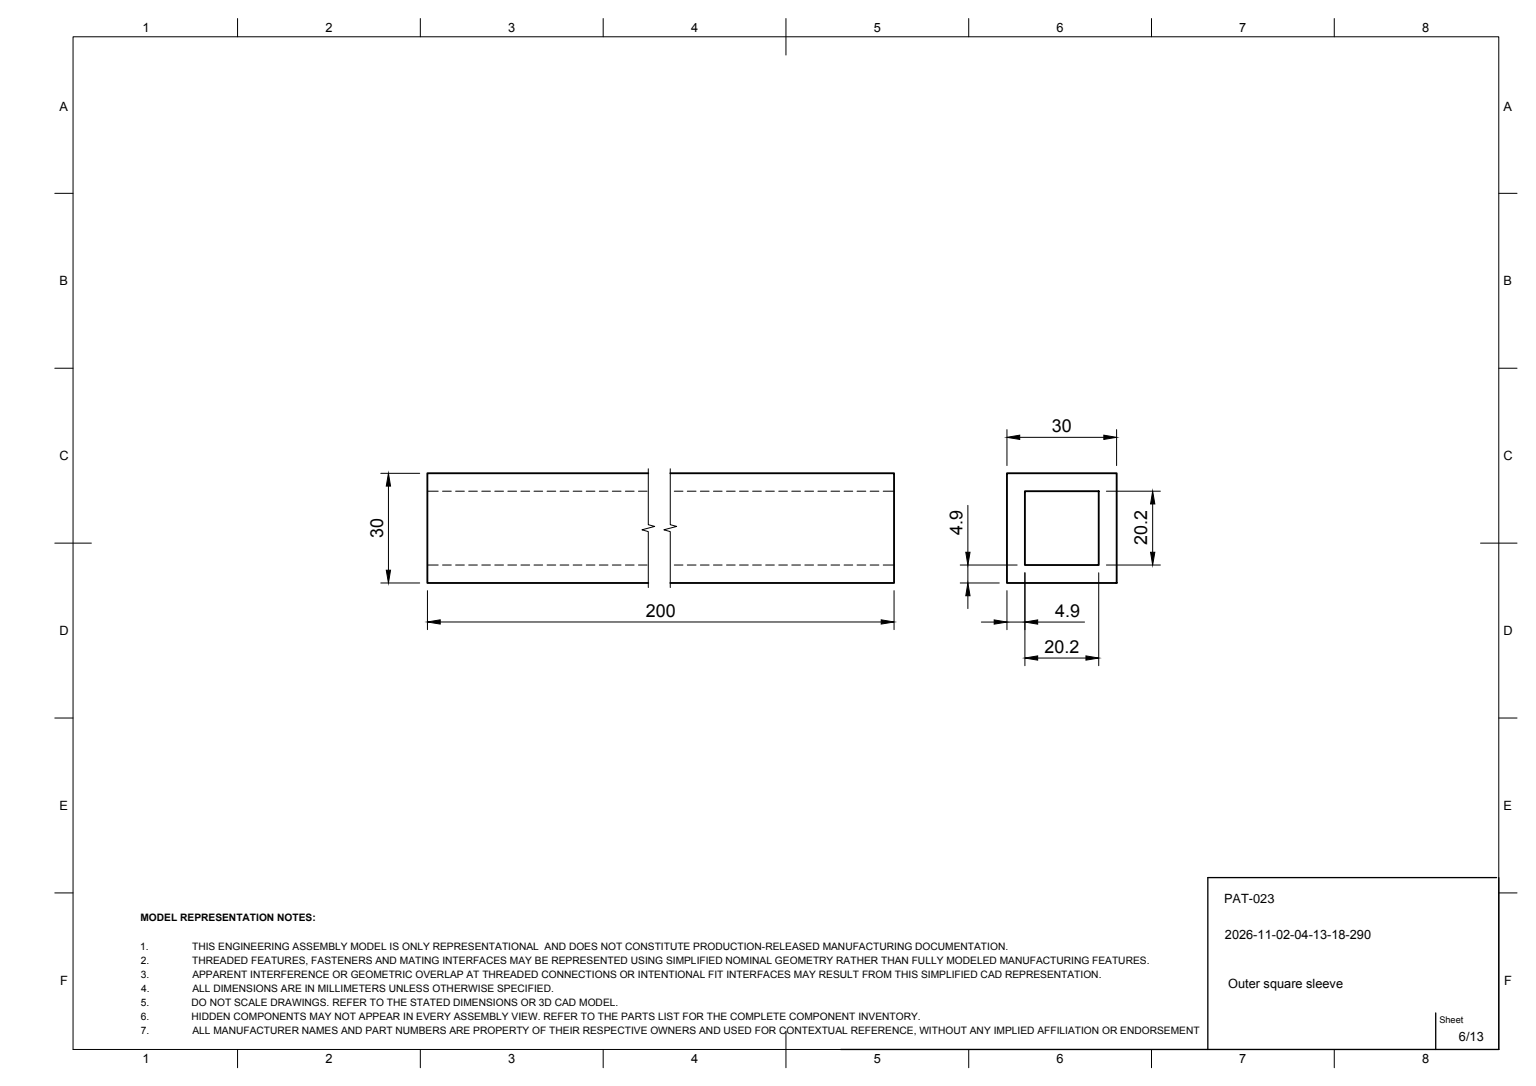
ISO-10303-21;
HEADER;
/* Generated by software containing ST-Developer
 * from STEP Tools, Inc. (www.steptools.com) 
 */

FILE_DESCRIPTION(
/* description */ ('PAT-023'),
/* implementation_level */ '2;1');

FILE_NAME(
/* name */ 'Outer square sleeve.step',
/* time_stamp */ '2026-10-29T15:47:46-07:00',
/* author */ (''),
/* organization */ (''),
/* preprocessor_version */ 'ST-DEVELOPER v20.2',
/* originating_system */ 'Autodesk Translation Framework v15.17.0.0',
/* authorisation */ '');

FILE_SCHEMA (('AUTOMOTIVE_DESIGN { 1 0 10303 214 3 1 1 }'));
ENDSEC;

DATA;
#10=MECHANICAL_DESIGN_GEOMETRIC_PRESENTATION_REPRESENTATION('',(#85),#3773);
#69=SHAPE_REPRESENTATION_RELATIONSHIP('SRR','None',#3816,#77);
#77=ADVANCED_BREP_SHAPE_REPRESENTATION('',(#93),#3764);
#85=STYLED_ITEM('',(#3939),#93);
#93=MANIFOLD_SOLID_BREP('Body1',#2238);
#102=FACE_BOUND('',#355,.T.);
#103=FACE_BOUND('',#357,.T.);
#121=PLANE('',#2347);
#122=PLANE('',#2348);
#123=PLANE('',#2349);
#124=PLANE('',#2350);
#125=PLANE('',#2351);
#126=PLANE('',#2352);
#127=PLANE('',#2353);
#128=PLANE('',#2354);
#129=PLANE('',#2355);
#130=PLANE('',#2356);
#225=FACE_OUTER_BOUND('',#346,.T.);
#226=FACE_OUTER_BOUND('',#347,.T.);
#227=FACE_OUTER_BOUND('',#348,.T.);
#228=FACE_OUTER_BOUND('',#349,.T.);
#229=FACE_OUTER_BOUND('',#350,.T.);
#230=FACE_OUTER_BOUND('',#351,.T.);
#231=FACE_OUTER_BOUND('',#352,.T.);
#232=FACE_OUTER_BOUND('',#353,.T.);
#233=FACE_OUTER_BOUND('',#354,.T.);
#234=FACE_OUTER_BOUND('',#356,.T.);
#346=EDGE_LOOP('',(#1547,#1548,#1549,#1550));
#347=EDGE_LOOP('',(#1551,#1552,#1553,#1554));
#348=EDGE_LOOP('',(#1555,#1556,#1557,#1558));
#349=EDGE_LOOP('',(#1559,#1560,#1561,#1562));
#350=EDGE_LOOP('',(#1563,#1564,#1565,#1566));
#351=EDGE_LOOP('',(#1567,#1568,#1569,#1570));
#352=EDGE_LOOP('',(#1571,#1572,#1573,#1574));
#353=EDGE_LOOP('',(#1575,#1576,#1577,#1578));
#354=EDGE_LOOP('',(#1579,#1580,#1581,#1582));
#355=EDGE_LOOP('',(#1583,#1584,#1585,#1586));
#356=EDGE_LOOP('',(#1587,#1588,#1589,#1590));
#357=EDGE_LOOP('',(#1591,#1592,#1593,#1594));
#484=LINE('',#3141,#748);
#485=LINE('',#3143,#749);
#486=LINE('',#3145,#750);
#487=LINE('',#3146,#751);
#488=LINE('',#3149,#752);
#489=LINE('',#3151,#753);
#490=LINE('',#3152,#754);
#491=LINE('',#3155,#755);
#492=LINE('',#3157,#756);
#493=LINE('',#3158,#757);
#494=LINE('',#3160,#758);
#495=LINE('',#3161,#759);
#496=LINE('',#3165,#760);
#497=LINE('',#3167,#761);
#498=LINE('',#3169,#762);
#499=LINE('',#3170,#763);
#500=LINE('',#3173,#764);
#501=LINE('',#3175,#765);
#502=LINE('',#3176,#766);
#503=LINE('',#3179,#767);
#504=LINE('',#3181,#768);
#505=LINE('',#3182,#769);
#506=LINE('',#3184,#770);
#507=LINE('',#3185,#771);
#748=VECTOR('',#2543,1.);
#749=VECTOR('',#2544,1.);
#750=VECTOR('',#2545,1.);
#751=VECTOR('',#2546,1.);
#752=VECTOR('',#2549,1.);
#753=VECTOR('',#2550,1.);
#754=VECTOR('',#2551,1.);
#755=VECTOR('',#2554,1.);
#756=VECTOR('',#2555,1.);
#757=VECTOR('',#2556,1.);
#758=VECTOR('',#2559,1.);
#759=VECTOR('',#2560,1.);
#760=VECTOR('',#2563,1.);
#761=VECTOR('',#2564,1.);
#762=VECTOR('',#2565,1.);
#763=VECTOR('',#2566,1.);
#764=VECTOR('',#2569,1.);
#765=VECTOR('',#2570,1.);
#766=VECTOR('',#2571,1.);
#767=VECTOR('',#2574,1.);
#768=VECTOR('',#2575,1.);
#769=VECTOR('',#2576,1.);
#770=VECTOR('',#2579,1.);
#771=VECTOR('',#2580,1.);
#1035=VERTEX_POINT('',#3139);
#1036=VERTEX_POINT('',#3140);
#1037=VERTEX_POINT('',#3142);
#1038=VERTEX_POINT('',#3144);
#1039=VERTEX_POINT('',#3148);
#1040=VERTEX_POINT('',#3150);
#1041=VERTEX_POINT('',#3154);
#1042=VERTEX_POINT('',#3156);
#1043=VERTEX_POINT('',#3163);
#1044=VERTEX_POINT('',#3164);
#1045=VERTEX_POINT('',#3166);
#1046=VERTEX_POINT('',#3168);
#1047=VERTEX_POINT('',#3172);
#1048=VERTEX_POINT('',#3174);
#1049=VERTEX_POINT('',#3178);
#1050=VERTEX_POINT('',#3180);
#1236=EDGE_CURVE('',#1035,#1036,#484,.T.);
#1237=EDGE_CURVE('',#1037,#1035,#485,.T.);
#1238=EDGE_CURVE('',#1038,#1037,#486,.T.);
#1239=EDGE_CURVE('',#1038,#1036,#487,.T.);
#1240=EDGE_CURVE('',#1036,#1039,#488,.T.);
#1241=EDGE_CURVE('',#1040,#1038,#489,.T.);
#1242=EDGE_CURVE('',#1040,#1039,#490,.T.);
#1243=EDGE_CURVE('',#1039,#1041,#491,.T.);
#1244=EDGE_CURVE('',#1042,#1040,#492,.T.);
#1245=EDGE_CURVE('',#1042,#1041,#493,.T.);
#1246=EDGE_CURVE('',#1041,#1035,#494,.T.);
#1247=EDGE_CURVE('',#1037,#1042,#495,.T.);
#1248=EDGE_CURVE('',#1043,#1044,#496,.T.);
#1249=EDGE_CURVE('',#1044,#1045,#497,.T.);
#1250=EDGE_CURVE('',#1046,#1045,#498,.T.);
#1251=EDGE_CURVE('',#1043,#1046,#499,.T.);
#1252=EDGE_CURVE('',#1047,#1043,#500,.T.);
#1253=EDGE_CURVE('',#1048,#1046,#501,.T.);
#1254=EDGE_CURVE('',#1047,#1048,#502,.T.);
#1255=EDGE_CURVE('',#1049,#1047,#503,.T.);
#1256=EDGE_CURVE('',#1050,#1048,#504,.T.);
#1257=EDGE_CURVE('',#1049,#1050,#505,.T.);
#1258=EDGE_CURVE('',#1044,#1049,#506,.T.);
#1259=EDGE_CURVE('',#1045,#1050,#507,.T.);
#1547=ORIENTED_EDGE('',*,*,#1236,.F.);
#1548=ORIENTED_EDGE('',*,*,#1237,.F.);
#1549=ORIENTED_EDGE('',*,*,#1238,.F.);
#1550=ORIENTED_EDGE('',*,*,#1239,.T.);
#1551=ORIENTED_EDGE('',*,*,#1240,.F.);
#1552=ORIENTED_EDGE('',*,*,#1239,.F.);
#1553=ORIENTED_EDGE('',*,*,#1241,.F.);
#1554=ORIENTED_EDGE('',*,*,#1242,.T.);
#1555=ORIENTED_EDGE('',*,*,#1243,.F.);
#1556=ORIENTED_EDGE('',*,*,#1242,.F.);
#1557=ORIENTED_EDGE('',*,*,#1244,.F.);
#1558=ORIENTED_EDGE('',*,*,#1245,.T.);
#1559=ORIENTED_EDGE('',*,*,#1246,.F.);
#1560=ORIENTED_EDGE('',*,*,#1245,.F.);
#1561=ORIENTED_EDGE('',*,*,#1247,.F.);
#1562=ORIENTED_EDGE('',*,*,#1237,.T.);
#1563=ORIENTED_EDGE('',*,*,#1248,.T.);
#1564=ORIENTED_EDGE('',*,*,#1249,.T.);
#1565=ORIENTED_EDGE('',*,*,#1250,.F.);
#1566=ORIENTED_EDGE('',*,*,#1251,.F.);
#1567=ORIENTED_EDGE('',*,*,#1252,.T.);
#1568=ORIENTED_EDGE('',*,*,#1251,.T.);
#1569=ORIENTED_EDGE('',*,*,#1253,.F.);
#1570=ORIENTED_EDGE('',*,*,#1254,.F.);
#1571=ORIENTED_EDGE('',*,*,#1255,.T.);
#1572=ORIENTED_EDGE('',*,*,#1254,.T.);
#1573=ORIENTED_EDGE('',*,*,#1256,.F.);
#1574=ORIENTED_EDGE('',*,*,#1257,.F.);
#1575=ORIENTED_EDGE('',*,*,#1258,.T.);
#1576=ORIENTED_EDGE('',*,*,#1257,.T.);
#1577=ORIENTED_EDGE('',*,*,#1259,.F.);
#1578=ORIENTED_EDGE('',*,*,#1249,.F.);
#1579=ORIENTED_EDGE('',*,*,#1259,.T.);
#1580=ORIENTED_EDGE('',*,*,#1256,.T.);
#1581=ORIENTED_EDGE('',*,*,#1253,.T.);
#1582=ORIENTED_EDGE('',*,*,#1250,.T.);
#1583=ORIENTED_EDGE('',*,*,#1243,.T.);
#1584=ORIENTED_EDGE('',*,*,#1246,.T.);
#1585=ORIENTED_EDGE('',*,*,#1236,.T.);
#1586=ORIENTED_EDGE('',*,*,#1240,.T.);
#1587=ORIENTED_EDGE('',*,*,#1258,.F.);
#1588=ORIENTED_EDGE('',*,*,#1248,.F.);
#1589=ORIENTED_EDGE('',*,*,#1252,.F.);
#1590=ORIENTED_EDGE('',*,*,#1255,.F.);
#1591=ORIENTED_EDGE('',*,*,#1244,.T.);
#1592=ORIENTED_EDGE('',*,*,#1241,.T.);
#1593=ORIENTED_EDGE('',*,*,#1238,.T.);
#1594=ORIENTED_EDGE('',*,*,#1247,.T.);
#2125=ADVANCED_FACE('',(#225),#121,.F.);
#2126=ADVANCED_FACE('',(#226),#122,.F.);
#2127=ADVANCED_FACE('',(#227),#123,.F.);
#2128=ADVANCED_FACE('',(#228),#124,.F.);
#2129=ADVANCED_FACE('',(#229),#125,.T.);
#2130=ADVANCED_FACE('',(#230),#126,.T.);
#2131=ADVANCED_FACE('',(#231),#127,.T.);
#2132=ADVANCED_FACE('',(#232),#128,.T.);
#2133=ADVANCED_FACE('',(#233,#102),#129,.T.);
#2134=ADVANCED_FACE('',(#234,#103),#130,.F.);
#2238=CLOSED_SHELL('',(#2125,#2126,#2127,#2128,#2129,#2130,#2131,#2132,
#2133,#2134));
#2346=AXIS2_PLACEMENT_3D('',#3137,#2539,#2540);
#2347=AXIS2_PLACEMENT_3D('',#3138,#2541,#2542);
#2348=AXIS2_PLACEMENT_3D('',#3147,#2547,#2548);
#2349=AXIS2_PLACEMENT_3D('',#3153,#2552,#2553);
#2350=AXIS2_PLACEMENT_3D('',#3159,#2557,#2558);
#2351=AXIS2_PLACEMENT_3D('',#3162,#2561,#2562);
#2352=AXIS2_PLACEMENT_3D('',#3171,#2567,#2568);
#2353=AXIS2_PLACEMENT_3D('',#3177,#2572,#2573);
#2354=AXIS2_PLACEMENT_3D('',#3183,#2577,#2578);
#2355=AXIS2_PLACEMENT_3D('',#3186,#2581,#2582);
#2356=AXIS2_PLACEMENT_3D('',#3187,#2583,#2584);
#2539=DIRECTION('axis',(0.,0.,1.));
#2540=DIRECTION('refdir',(1.,0.,0.));
#2541=DIRECTION('center_axis',(0.,-1.,0.));
#2542=DIRECTION('ref_axis',(1.,0.,0.));
#2543=DIRECTION('',(-1.,0.,0.));
#2544=DIRECTION('',(0.,0.,1.));
#2545=DIRECTION('',(1.,0.,0.));
#2546=DIRECTION('',(0.,0.,1.));
#2547=DIRECTION('center_axis',(-1.,0.,0.));
#2548=DIRECTION('ref_axis',(0.,-1.,0.));
#2549=DIRECTION('',(0.,1.,0.));
#2550=DIRECTION('',(0.,-1.,0.));
#2551=DIRECTION('',(0.,0.,1.));
#2552=DIRECTION('center_axis',(0.,1.,0.));
#2553=DIRECTION('ref_axis',(-1.,0.,0.));
#2554=DIRECTION('',(1.,0.,0.));
#2555=DIRECTION('',(-1.,0.,0.));
#2556=DIRECTION('',(0.,0.,1.));
#2557=DIRECTION('center_axis',(1.,0.,0.));
#2558=DIRECTION('ref_axis',(0.,1.,0.));
#2559=DIRECTION('',(0.,-1.,0.));
#2560=DIRECTION('',(0.,1.,0.));
#2561=DIRECTION('center_axis',(0.,1.,0.));
#2562=DIRECTION('ref_axis',(-1.,0.,0.));
#2563=DIRECTION('',(-1.,0.,0.));
#2564=DIRECTION('',(0.,0.,1.));
#2565=DIRECTION('',(-1.,0.,0.));
#2566=DIRECTION('',(0.,0.,1.));
#2567=DIRECTION('center_axis',(1.,0.,0.));
#2568=DIRECTION('ref_axis',(0.,1.,0.));
#2569=DIRECTION('',(0.,1.,0.));
#2570=DIRECTION('',(0.,1.,0.));
#2571=DIRECTION('',(0.,0.,1.));
#2572=DIRECTION('center_axis',(0.,-1.,0.));
#2573=DIRECTION('ref_axis',(1.,0.,0.));
#2574=DIRECTION('',(1.,0.,0.));
#2575=DIRECTION('',(1.,0.,0.));
#2576=DIRECTION('',(0.,0.,1.));
#2577=DIRECTION('center_axis',(-1.,0.,0.));
#2578=DIRECTION('ref_axis',(0.,-1.,0.));
#2579=DIRECTION('',(0.,-1.,0.));
#2580=DIRECTION('',(0.,-1.,0.));
#2581=DIRECTION('center_axis',(0.,0.,1.));
#2582=DIRECTION('ref_axis',(1.,0.,0.));
#2583=DIRECTION('center_axis',(0.,0.,1.));
#2584=DIRECTION('ref_axis',(1.,0.,0.));
#3137=CARTESIAN_POINT('',(0.,0.,0.));
#3138=CARTESIAN_POINT('Origin',(-1.01,-1.01,6.9));
#3139=CARTESIAN_POINT('',(1.01,-1.01,27.));
#3140=CARTESIAN_POINT('',(-1.01,-1.01,27.));
#3141=CARTESIAN_POINT('',(-0.505,-1.01,27.));
#3142=CARTESIAN_POINT('',(1.01,-1.01,7.));
#3143=CARTESIAN_POINT('',(1.01,-1.01,6.9));
#3144=CARTESIAN_POINT('',(-1.01,-1.01,7.));
#3145=CARTESIAN_POINT('',(-0.505,-1.01,7.));
#3146=CARTESIAN_POINT('',(-1.01,-1.01,6.9));
#3147=CARTESIAN_POINT('Origin',(-1.01,1.01,6.9));
#3148=CARTESIAN_POINT('',(-1.01,1.01,27.));
#3149=CARTESIAN_POINT('',(-1.01,0.505,27.));
#3150=CARTESIAN_POINT('',(-1.01,1.01,7.));
#3151=CARTESIAN_POINT('',(-1.01,0.505,7.));
#3152=CARTESIAN_POINT('',(-1.01,1.01,6.9));
#3153=CARTESIAN_POINT('Origin',(1.01,1.01,6.9));
#3154=CARTESIAN_POINT('',(1.01,1.01,27.));
#3155=CARTESIAN_POINT('',(0.505,1.01,27.));
#3156=CARTESIAN_POINT('',(1.01,1.01,7.));
#3157=CARTESIAN_POINT('',(0.505,1.01,7.));
#3158=CARTESIAN_POINT('',(1.01,1.01,6.9));
#3159=CARTESIAN_POINT('Origin',(1.01,-1.01,6.9));
#3160=CARTESIAN_POINT('',(1.01,-0.505,27.));
#3161=CARTESIAN_POINT('',(1.01,-0.505,7.));
#3162=CARTESIAN_POINT('Origin',(1.5,1.5,7.));
#3163=CARTESIAN_POINT('',(1.5,1.5,7.));
#3164=CARTESIAN_POINT('',(-1.5,1.5,7.));
#3165=CARTESIAN_POINT('',(1.5,1.5,7.));
#3166=CARTESIAN_POINT('',(-1.5,1.5,27.));
#3167=CARTESIAN_POINT('',(-1.5,1.5,7.));
#3168=CARTESIAN_POINT('',(1.5,1.5,27.));
#3169=CARTESIAN_POINT('',(1.5,1.5,27.));
#3170=CARTESIAN_POINT('',(1.5,1.5,7.));
#3171=CARTESIAN_POINT('Origin',(1.5,-1.5,7.));
#3172=CARTESIAN_POINT('',(1.5,-1.5,7.));
#3173=CARTESIAN_POINT('',(1.5,-1.5,7.));
#3174=CARTESIAN_POINT('',(1.5,-1.5,27.));
#3175=CARTESIAN_POINT('',(1.5,-1.5,27.));
#3176=CARTESIAN_POINT('',(1.5,-1.5,7.));
#3177=CARTESIAN_POINT('Origin',(-1.5,-1.5,7.));
#3178=CARTESIAN_POINT('',(-1.5,-1.5,7.));
#3179=CARTESIAN_POINT('',(-1.5,-1.5,7.));
#3180=CARTESIAN_POINT('',(-1.5,-1.5,27.));
#3181=CARTESIAN_POINT('',(-1.5,-1.5,27.));
#3182=CARTESIAN_POINT('',(-1.5,-1.5,7.));
#3183=CARTESIAN_POINT('Origin',(-1.5,1.5,7.));
#3184=CARTESIAN_POINT('',(-1.5,1.5,7.));
#3185=CARTESIAN_POINT('',(-1.5,1.5,27.));
#3186=CARTESIAN_POINT('Origin',(0.,0.,27.));
#3187=CARTESIAN_POINT('Origin',(0.,0.,7.));
#3751=UNCERTAINTY_MEASURE_WITH_UNIT(LENGTH_MEASURE(0.001),#3774,
'DISTANCE_ACCURACY_VALUE',
'Maximum model space distance between geometric entities at asserted c
onnectivities');
#3760=UNCERTAINTY_MEASURE_WITH_UNIT(LENGTH_MEASURE(0.001),#3774,
'DISTANCE_ACCURACY_VALUE',
'Maximum model space distance between geometric entities at asserted c
onnectivities');
#3764=(
GEOMETRIC_REPRESENTATION_CONTEXT(3)
GLOBAL_UNCERTAINTY_ASSIGNED_CONTEXT((#3751))
GLOBAL_UNIT_ASSIGNED_CONTEXT((#3774,#3776,#3777))
REPRESENTATION_CONTEXT('','3D')
);
#3773=(
GEOMETRIC_REPRESENTATION_CONTEXT(3)
GLOBAL_UNCERTAINTY_ASSIGNED_CONTEXT((#3760))
GLOBAL_UNIT_ASSIGNED_CONTEXT((#3774,#3776,#3777))
REPRESENTATION_CONTEXT('','3D')
);
#3774=(
LENGTH_UNIT()
NAMED_UNIT(*)
SI_UNIT(.CENTI.,.METRE.)
);
#3776=(
NAMED_UNIT(*)
PLANE_ANGLE_UNIT()
SI_UNIT($,.RADIAN.)
);
#3777=(
NAMED_UNIT(*)
SI_UNIT($,.STERADIAN.)
SOLID_ANGLE_UNIT()
);
#3781=SHAPE_DEFINITION_REPRESENTATION(#3793,#3816);
#3793=PRODUCT_DEFINITION_SHAPE('',$,#3829);
#3816=SHAPE_REPRESENTATION('',(#2346),#3764);
#3825=PRODUCT_DEFINITION_CONTEXT('part definition',#3863,'design');
#3829=PRODUCT_DEFINITION('Outer square sleeve',
'Outer square sleeve',#3841,#3825);
#3841=PRODUCT_DEFINITION_FORMATION('',$,#3868);
#3863=APPLICATION_CONTEXT(
'Core Data for Automotive Mechanical Design Process');
#3864=PRODUCT_CONTEXT('part definition',#3863,'mechanical');
#3868=PRODUCT('Outer square sleeve','Outer square sleeve',
'Outer square sleeve',(#3864));
#3933=COLOUR_RGB('Sky Blue',0.24,0.69,0.87);
#3934=FILL_AREA_STYLE_COLOUR('',#3933);
#3935=FILL_AREA_STYLE('',(#3934));
#3936=SURFACE_STYLE_FILL_AREA(#3935);
#3937=SURFACE_SIDE_STYLE('',(#3936));
#3938=SURFACE_STYLE_USAGE(.BOTH.,#3937);
#3939=PRESENTATION_STYLE_ASSIGNMENT((#3938));
ENDSEC;
END-ISO-10303-21;
